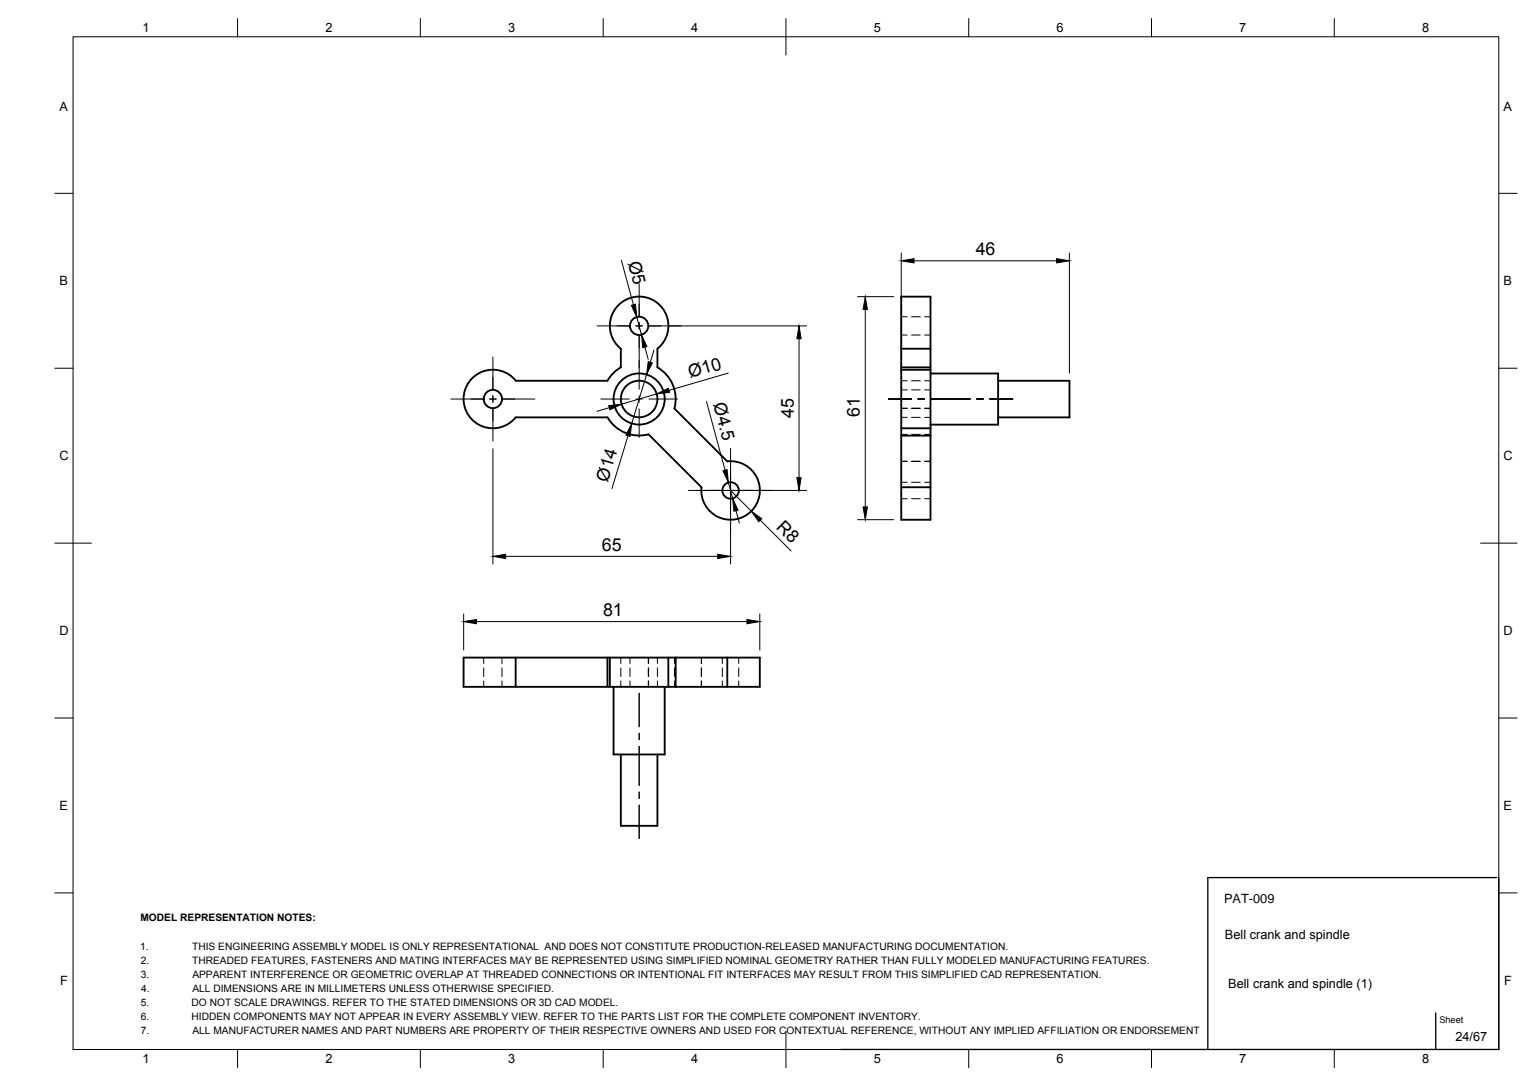
ISO-10303-21;
HEADER;
/* Generated by software containing ST-Developer
 * from STEP Tools, Inc. (www.steptools.com) 
 */

FILE_DESCRIPTION(
/* description */ ('Bell-crank linkage with push rods'),
/* implementation_level */ '2;1');

FILE_NAME(
/* name */ 'Bell crank and spindle (1).step',
/* time_stamp */ '2026-10-28T03:25:15-07:00',
/* author */ (''),
/* organization */ (''),
/* preprocessor_version */ 'ST-DEVELOPER v20.2',
/* originating_system */ 'Autodesk Translation Framework v15.17.0.0',
/* authorisation */ '');

FILE_SCHEMA (('AUTOMOTIVE_DESIGN { 1 0 10303 214 3 1 1 }'));
ENDSEC;

DATA;
#10=MECHANICAL_DESIGN_GEOMETRIC_PRESENTATION_REPRESENTATION('',(#629),#16678);
#513=SHAPE_REPRESENTATION_RELATIONSHIP('SRR','None',#16931,#567);
#567=ADVANCED_BREP_SHAPE_REPRESENTATION('',(#690),#16636);
#629=STYLED_ITEM('',(#17284),#690);
#690=MANIFOLD_SOLID_BREP('Body1',#8820);
#823=FACE_BOUND('',#2103,.T.);
#824=FACE_BOUND('',#2104,.T.);
#825=FACE_BOUND('',#2105,.T.);
#826=FACE_BOUND('',#2112,.T.);
#827=FACE_BOUND('',#2113,.T.);
#828=FACE_BOUND('',#2114,.T.);
#829=FACE_BOUND('',#2115,.T.);
#830=FACE_BOUND('',#2122,.T.);
#1082=PLANE('',#9961);
#1083=PLANE('',#9962);
#1084=PLANE('',#9968);
#1085=PLANE('',#9975);
#1086=PLANE('',#9976);
#1087=PLANE('',#9980);
#1088=PLANE('',#9982);
#1089=PLANE('',#9983);
#1090=PLANE('',#9985);
#1091=PLANE('',#9991);
#1477=FACE_OUTER_BOUND('',#2097,.T.);
#1478=FACE_OUTER_BOUND('',#2098,.T.);
#1479=FACE_OUTER_BOUND('',#2099,.T.);
#1480=FACE_OUTER_BOUND('',#2100,.T.);
#1481=FACE_OUTER_BOUND('',#2101,.T.);
#1482=FACE_OUTER_BOUND('',#2102,.T.);
#1483=FACE_OUTER_BOUND('',#2106,.T.);
#1484=FACE_OUTER_BOUND('',#2107,.T.);
#1485=FACE_OUTER_BOUND('',#2108,.T.);
#1486=FACE_OUTER_BOUND('',#2109,.T.);
#1487=FACE_OUTER_BOUND('',#2110,.T.);
#1488=FACE_OUTER_BOUND('',#2111,.T.);
#1489=FACE_OUTER_BOUND('',#2116,.T.);
#1490=FACE_OUTER_BOUND('',#2117,.T.);
#1491=FACE_OUTER_BOUND('',#2118,.T.);
#1492=FACE_OUTER_BOUND('',#2119,.T.);
#1493=FACE_OUTER_BOUND('',#2120,.T.);
#1494=FACE_OUTER_BOUND('',#2121,.T.);
#1495=FACE_OUTER_BOUND('',#2123,.T.);
#1496=FACE_OUTER_BOUND('',#2124,.T.);
#1497=FACE_OUTER_BOUND('',#2125,.T.);
#2097=EDGE_LOOP('',(#6947,#6948,#6949,#6950));
#2098=EDGE_LOOP('',(#6951,#6952,#6953,#6954));
#2099=EDGE_LOOP('',(#6955,#6956,#6957,#6958));
#2100=EDGE_LOOP('',(#6959,#6960,#6961,#6962));
#2101=EDGE_LOOP('',(#6963,#6964,#6965,#6966));
#2102=EDGE_LOOP('',(#6967,#6968,#6969,#6970,#6971,#6972,#6973,#6974,#6975,
#6976,#6977,#6978));
#2103=EDGE_LOOP('',(#6979));
#2104=EDGE_LOOP('',(#6980));
#2105=EDGE_LOOP('',(#6981));
#2106=EDGE_LOOP('',(#6982,#6983,#6984,#6985));
#2107=EDGE_LOOP('',(#6986,#6987,#6988,#6989));
#2108=EDGE_LOOP('',(#6990,#6991,#6992,#6993));
#2109=EDGE_LOOP('',(#6994,#6995,#6996,#6997));
#2110=EDGE_LOOP('',(#6998,#6999,#7000,#7001));
#2111=EDGE_LOOP('',(#7002,#7003,#7004,#7005,#7006,#7007,#7008,#7009,#7010,
#7011,#7012,#7013));
#2112=EDGE_LOOP('',(#7014));
#2113=EDGE_LOOP('',(#7015));
#2114=EDGE_LOOP('',(#7016));
#2115=EDGE_LOOP('',(#7017));
#2116=EDGE_LOOP('',(#7018,#7019,#7020,#7021));
#2117=EDGE_LOOP('',(#7022,#7023,#7024,#7025));
#2118=EDGE_LOOP('',(#7026,#7027,#7028,#7029));
#2119=EDGE_LOOP('',(#7030,#7031,#7032,#7033));
#2120=EDGE_LOOP('',(#7034,#7035,#7036,#7037));
#2121=EDGE_LOOP('',(#7038));
#2122=EDGE_LOOP('',(#7039));
#2123=EDGE_LOOP('',(#7040,#7041,#7042,#7043));
#2124=EDGE_LOOP('',(#7044,#7045,#7046,#7047));
#2125=EDGE_LOOP('',(#7048));
#2778=LINE('',#15134,#3327);
#2779=LINE('',#15140,#3328);
#2780=LINE('',#15146,#3329);
#2781=LINE('',#15151,#3330);
#2782=LINE('',#15155,#3331);
#2783=LINE('',#15159,#3332);
#2784=LINE('',#15161,#3333);
#2785=LINE('',#15162,#3334);
#2786=LINE('',#15165,#3335);
#2787=LINE('',#15169,#3336);
#2788=LINE('',#15173,#3337);
#2789=LINE('',#15177,#3338);
#2790=LINE('',#15181,#3339);
#2791=LINE('',#15185,#3340);
#2792=LINE('',#15186,#3341);
#2793=LINE('',#15189,#3342);
#2794=LINE('',#15194,#3343);
#2795=LINE('',#15197,#3344);
#2796=LINE('',#15199,#3345);
#2797=LINE('',#15203,#3346);
#2798=LINE('',#15204,#3347);
#2799=LINE('',#15207,#3348);
#2800=LINE('',#15211,#3349);
#2801=LINE('',#15213,#3350);
#2802=LINE('',#15218,#3351);
#2803=LINE('',#15219,#3352);
#2804=LINE('',#15221,#3353);
#2805=LINE('',#15230,#3354);
#2806=LINE('',#15233,#3355);
#3327=VECTOR('',#11870,0.25);
#3328=VECTOR('',#11877,0.25);
#3329=VECTOR('',#11884,0.225);
#3330=VECTOR('',#11889,1.);
#3331=VECTOR('',#11892,1.);
#3332=VECTOR('',#11897,1.);
#3333=VECTOR('',#11898,1.);
#3334=VECTOR('',#11899,1.);
#3335=VECTOR('',#11902,1.);
#3336=VECTOR('',#11905,1.);
#3337=VECTOR('',#11908,1.);
#3338=VECTOR('',#11911,1.);
#3339=VECTOR('',#11914,1.);
#3340=VECTOR('',#11919,1.);
#3341=VECTOR('',#11920,1.);
#3342=VECTOR('',#11923,1.);
#3343=VECTOR('',#11930,1.);
#3344=VECTOR('',#11933,1.);
#3345=VECTOR('',#11934,1.);
#3346=VECTOR('',#11939,1.);
#3347=VECTOR('',#11940,1.);
#3348=VECTOR('',#11943,1.);
#3349=VECTOR('',#11946,1.);
#3350=VECTOR('',#11949,1.);
#3351=VECTOR('',#11956,1.);
#3352=VECTOR('',#11957,1.);
#3353=VECTOR('',#11960,1.);
#3354=VECTOR('',#11973,0.7);
#3355=VECTOR('',#11976,0.5);
#3868=CIRCLE('',#9950,0.25);
#3869=CIRCLE('',#9951,0.25);
#3870=CIRCLE('',#9953,0.25);
#3871=CIRCLE('',#9954,0.25);
#3872=CIRCLE('',#9956,0.225);
#3873=CIRCLE('',#9957,0.225);
#3874=CIRCLE('',#9959,0.8);
#3875=CIRCLE('',#9960,0.8);
#3876=CIRCLE('',#9963,1.);
#3877=CIRCLE('',#9964,0.8);
#3878=CIRCLE('',#9965,1.);
#3879=CIRCLE('',#9966,0.8);
#3880=CIRCLE('',#9967,1.);
#3881=CIRCLE('',#9970,1.);
#3882=CIRCLE('',#9972,1.);
#3883=CIRCLE('',#9974,0.8);
#3884=CIRCLE('',#9977,0.8);
#3885=CIRCLE('',#9978,1.);
#3886=CIRCLE('',#9979,0.7);
#3887=CIRCLE('',#9986,0.7);
#3888=CIRCLE('',#9987,0.5);
#3889=CIRCLE('',#9990,0.5);
#4462=VERTEX_POINT('',#15131);
#4463=VERTEX_POINT('',#15133);
#4464=VERTEX_POINT('',#15137);
#4465=VERTEX_POINT('',#15139);
#4466=VERTEX_POINT('',#15143);
#4467=VERTEX_POINT('',#15145);
#4468=VERTEX_POINT('',#15149);
#4469=VERTEX_POINT('',#15150);
#4470=VERTEX_POINT('',#15152);
#4471=VERTEX_POINT('',#15154);
#4472=VERTEX_POINT('',#15158);
#4473=VERTEX_POINT('',#15160);
#4474=VERTEX_POINT('',#15164);
#4475=VERTEX_POINT('',#15166);
#4476=VERTEX_POINT('',#15168);
#4477=VERTEX_POINT('',#15170);
#4478=VERTEX_POINT('',#15172);
#4479=VERTEX_POINT('',#15174);
#4480=VERTEX_POINT('',#15176);
#4481=VERTEX_POINT('',#15178);
#4482=VERTEX_POINT('',#15180);
#4483=VERTEX_POINT('',#15184);
#4484=VERTEX_POINT('',#15188);
#4485=VERTEX_POINT('',#15192);
#4486=VERTEX_POINT('',#15196);
#4487=VERTEX_POINT('',#15198);
#4488=VERTEX_POINT('',#15202);
#4489=VERTEX_POINT('',#15206);
#4490=VERTEX_POINT('',#15208);
#4491=VERTEX_POINT('',#15210);
#4492=VERTEX_POINT('',#15214);
#4493=VERTEX_POINT('',#15225);
#4494=VERTEX_POINT('',#15227);
#4495=VERTEX_POINT('',#15232);
#5351=EDGE_CURVE('',#4462,#4462,#3868,.T.);
#5352=EDGE_CURVE('',#4462,#4463,#2778,.T.);
#5353=EDGE_CURVE('',#4463,#4463,#3869,.T.);
#5354=EDGE_CURVE('',#4464,#4464,#3870,.T.);
#5355=EDGE_CURVE('',#4464,#4465,#2779,.T.);
#5356=EDGE_CURVE('',#4465,#4465,#3871,.T.);
#5357=EDGE_CURVE('',#4466,#4466,#3872,.T.);
#5358=EDGE_CURVE('',#4466,#4467,#2780,.T.);
#5359=EDGE_CURVE('',#4467,#4467,#3873,.T.);
#5360=EDGE_CURVE('',#4468,#4469,#2781,.T.);
#5361=EDGE_CURVE('',#4468,#4470,#3874,.T.);
#5362=EDGE_CURVE('',#4471,#4470,#2782,.T.);
#5363=EDGE_CURVE('',#4469,#4471,#3875,.T.);
#5364=EDGE_CURVE('',#4472,#4469,#2783,.T.);
#5365=EDGE_CURVE('',#4473,#4472,#2784,.T.);
#5366=EDGE_CURVE('',#4468,#4473,#2785,.T.);
#5367=EDGE_CURVE('',#4471,#4474,#2786,.T.);
#5368=EDGE_CURVE('',#4474,#4475,#3876,.T.);
#5369=EDGE_CURVE('',#4475,#4476,#2787,.T.);
#5370=EDGE_CURVE('',#4476,#4477,#3877,.T.);
#5371=EDGE_CURVE('',#4477,#4478,#2788,.T.);
#5372=EDGE_CURVE('',#4478,#4479,#3878,.T.);
#5373=EDGE_CURVE('',#4479,#4480,#2789,.T.);
#5374=EDGE_CURVE('',#4480,#4481,#3879,.T.);
#5375=EDGE_CURVE('',#4481,#4482,#2790,.T.);
#5376=EDGE_CURVE('',#4482,#4472,#3880,.T.);
#5377=EDGE_CURVE('',#4483,#4470,#2791,.T.);
#5378=EDGE_CURVE('',#4474,#4483,#2792,.T.);
#5379=EDGE_CURVE('',#4482,#4484,#2793,.T.);
#5380=EDGE_CURVE('',#4484,#4473,#3881,.T.);
#5381=EDGE_CURVE('',#4483,#4485,#3882,.T.);
#5382=EDGE_CURVE('',#4485,#4475,#2794,.T.);
#5383=EDGE_CURVE('',#4477,#4486,#2795,.T.);
#5384=EDGE_CURVE('',#4487,#4476,#2796,.T.);
#5385=EDGE_CURVE('',#4487,#4486,#3883,.T.);
#5386=EDGE_CURVE('',#4488,#4486,#2797,.T.);
#5387=EDGE_CURVE('',#4478,#4488,#2798,.T.);
#5388=EDGE_CURVE('',#4484,#4489,#2799,.T.);
#5389=EDGE_CURVE('',#4490,#4489,#3884,.T.);
#5390=EDGE_CURVE('',#4490,#4491,#2800,.T.);
#5391=EDGE_CURVE('',#4488,#4491,#3885,.T.);
#5392=EDGE_CURVE('',#4487,#4485,#2801,.T.);
#5393=EDGE_CURVE('',#4492,#4492,#3886,.T.);
#5394=EDGE_CURVE('',#4490,#4480,#2802,.T.);
#5395=EDGE_CURVE('',#4481,#4489,#2803,.T.);
#5396=EDGE_CURVE('',#4491,#4479,#2804,.T.);
#5397=EDGE_CURVE('',#4493,#4493,#3887,.T.);
#5398=EDGE_CURVE('',#4494,#4494,#3888,.T.);
#5399=EDGE_CURVE('',#4492,#4493,#2805,.T.);
#5400=EDGE_CURVE('',#4494,#4495,#2806,.T.);
#5401=EDGE_CURVE('',#4495,#4495,#3889,.T.);
#6947=ORIENTED_EDGE('',*,*,#5351,.F.);
#6948=ORIENTED_EDGE('',*,*,#5352,.T.);
#6949=ORIENTED_EDGE('',*,*,#5353,.F.);
#6950=ORIENTED_EDGE('',*,*,#5352,.F.);
#6951=ORIENTED_EDGE('',*,*,#5354,.F.);
#6952=ORIENTED_EDGE('',*,*,#5355,.T.);
#6953=ORIENTED_EDGE('',*,*,#5356,.F.);
#6954=ORIENTED_EDGE('',*,*,#5355,.F.);
#6955=ORIENTED_EDGE('',*,*,#5357,.F.);
#6956=ORIENTED_EDGE('',*,*,#5358,.T.);
#6957=ORIENTED_EDGE('',*,*,#5359,.F.);
#6958=ORIENTED_EDGE('',*,*,#5358,.F.);
#6959=ORIENTED_EDGE('',*,*,#5360,.F.);
#6960=ORIENTED_EDGE('',*,*,#5361,.T.);
#6961=ORIENTED_EDGE('',*,*,#5362,.F.);
#6962=ORIENTED_EDGE('',*,*,#5363,.F.);
#6963=ORIENTED_EDGE('',*,*,#5360,.T.);
#6964=ORIENTED_EDGE('',*,*,#5364,.F.);
#6965=ORIENTED_EDGE('',*,*,#5365,.F.);
#6966=ORIENTED_EDGE('',*,*,#5366,.F.);
#6967=ORIENTED_EDGE('',*,*,#5363,.T.);
#6968=ORIENTED_EDGE('',*,*,#5367,.T.);
#6969=ORIENTED_EDGE('',*,*,#5368,.T.);
#6970=ORIENTED_EDGE('',*,*,#5369,.T.);
#6971=ORIENTED_EDGE('',*,*,#5370,.T.);
#6972=ORIENTED_EDGE('',*,*,#5371,.T.);
#6973=ORIENTED_EDGE('',*,*,#5372,.T.);
#6974=ORIENTED_EDGE('',*,*,#5373,.T.);
#6975=ORIENTED_EDGE('',*,*,#5374,.T.);
#6976=ORIENTED_EDGE('',*,*,#5375,.T.);
#6977=ORIENTED_EDGE('',*,*,#5376,.T.);
#6978=ORIENTED_EDGE('',*,*,#5364,.T.);
#6979=ORIENTED_EDGE('',*,*,#5353,.T.);
#6980=ORIENTED_EDGE('',*,*,#5356,.T.);
#6981=ORIENTED_EDGE('',*,*,#5359,.T.);
#6982=ORIENTED_EDGE('',*,*,#5362,.T.);
#6983=ORIENTED_EDGE('',*,*,#5377,.F.);
#6984=ORIENTED_EDGE('',*,*,#5378,.F.);
#6985=ORIENTED_EDGE('',*,*,#5367,.F.);
#6986=ORIENTED_EDGE('',*,*,#5365,.T.);
#6987=ORIENTED_EDGE('',*,*,#5376,.F.);
#6988=ORIENTED_EDGE('',*,*,#5379,.T.);
#6989=ORIENTED_EDGE('',*,*,#5380,.T.);
#6990=ORIENTED_EDGE('',*,*,#5378,.T.);
#6991=ORIENTED_EDGE('',*,*,#5381,.T.);
#6992=ORIENTED_EDGE('',*,*,#5382,.T.);
#6993=ORIENTED_EDGE('',*,*,#5368,.F.);
#6994=ORIENTED_EDGE('',*,*,#5383,.F.);
#6995=ORIENTED_EDGE('',*,*,#5370,.F.);
#6996=ORIENTED_EDGE('',*,*,#5384,.F.);
#6997=ORIENTED_EDGE('',*,*,#5385,.T.);
#6998=ORIENTED_EDGE('',*,*,#5383,.T.);
#6999=ORIENTED_EDGE('',*,*,#5386,.F.);
#7000=ORIENTED_EDGE('',*,*,#5387,.F.);
#7001=ORIENTED_EDGE('',*,*,#5371,.F.);
#7002=ORIENTED_EDGE('',*,*,#5366,.T.);
#7003=ORIENTED_EDGE('',*,*,#5380,.F.);
#7004=ORIENTED_EDGE('',*,*,#5388,.T.);
#7005=ORIENTED_EDGE('',*,*,#5389,.F.);
#7006=ORIENTED_EDGE('',*,*,#5390,.T.);
#7007=ORIENTED_EDGE('',*,*,#5391,.F.);
#7008=ORIENTED_EDGE('',*,*,#5386,.T.);
#7009=ORIENTED_EDGE('',*,*,#5385,.F.);
#7010=ORIENTED_EDGE('',*,*,#5392,.T.);
#7011=ORIENTED_EDGE('',*,*,#5381,.F.);
#7012=ORIENTED_EDGE('',*,*,#5377,.T.);
#7013=ORIENTED_EDGE('',*,*,#5361,.F.);
#7014=ORIENTED_EDGE('',*,*,#5351,.T.);
#7015=ORIENTED_EDGE('',*,*,#5354,.T.);
#7016=ORIENTED_EDGE('',*,*,#5357,.T.);
#7017=ORIENTED_EDGE('',*,*,#5393,.T.);
#7018=ORIENTED_EDGE('',*,*,#5384,.T.);
#7019=ORIENTED_EDGE('',*,*,#5369,.F.);
#7020=ORIENTED_EDGE('',*,*,#5382,.F.);
#7021=ORIENTED_EDGE('',*,*,#5392,.F.);
#7022=ORIENTED_EDGE('',*,*,#5394,.F.);
#7023=ORIENTED_EDGE('',*,*,#5389,.T.);
#7024=ORIENTED_EDGE('',*,*,#5395,.F.);
#7025=ORIENTED_EDGE('',*,*,#5374,.F.);
#7026=ORIENTED_EDGE('',*,*,#5394,.T.);
#7027=ORIENTED_EDGE('',*,*,#5373,.F.);
#7028=ORIENTED_EDGE('',*,*,#5396,.F.);
#7029=ORIENTED_EDGE('',*,*,#5390,.F.);
#7030=ORIENTED_EDGE('',*,*,#5395,.T.);
#7031=ORIENTED_EDGE('',*,*,#5388,.F.);
#7032=ORIENTED_EDGE('',*,*,#5379,.F.);
#7033=ORIENTED_EDGE('',*,*,#5375,.F.);
#7034=ORIENTED_EDGE('',*,*,#5387,.T.);
#7035=ORIENTED_EDGE('',*,*,#5391,.T.);
#7036=ORIENTED_EDGE('',*,*,#5396,.T.);
#7037=ORIENTED_EDGE('',*,*,#5372,.F.);
#7038=ORIENTED_EDGE('',*,*,#5397,.F.);
#7039=ORIENTED_EDGE('',*,*,#5398,.F.);
#7040=ORIENTED_EDGE('',*,*,#5393,.F.);
#7041=ORIENTED_EDGE('',*,*,#5399,.T.);
#7042=ORIENTED_EDGE('',*,*,#5397,.T.);
#7043=ORIENTED_EDGE('',*,*,#5399,.F.);
#7044=ORIENTED_EDGE('',*,*,#5398,.T.);
#7045=ORIENTED_EDGE('',*,*,#5400,.T.);
#7046=ORIENTED_EDGE('',*,*,#5401,.T.);
#7047=ORIENTED_EDGE('',*,*,#5400,.F.);
#7048=ORIENTED_EDGE('',*,*,#5401,.F.);
#8153=CYLINDRICAL_SURFACE('',#9949,0.25);
#8154=CYLINDRICAL_SURFACE('',#9952,0.25);
#8155=CYLINDRICAL_SURFACE('',#9955,0.225);
#8156=CYLINDRICAL_SURFACE('',#9958,0.8);
#8157=CYLINDRICAL_SURFACE('',#9969,1.);
#8158=CYLINDRICAL_SURFACE('',#9971,1.);
#8159=CYLINDRICAL_SURFACE('',#9973,0.8);
#8160=CYLINDRICAL_SURFACE('',#9981,0.8);
#8161=CYLINDRICAL_SURFACE('',#9984,1.);
#8162=CYLINDRICAL_SURFACE('',#9988,0.7);
#8163=CYLINDRICAL_SURFACE('',#9989,0.5);
#8502=ADVANCED_FACE('',(#1477),#8153,.F.);
#8503=ADVANCED_FACE('',(#1478),#8154,.F.);
#8504=ADVANCED_FACE('',(#1479),#8155,.F.);
#8505=ADVANCED_FACE('',(#1480),#8156,.T.);
#8506=ADVANCED_FACE('',(#1481),#1082,.T.);
#8507=ADVANCED_FACE('',(#1482,#823,#824,#825),#1083,.T.);
#8508=ADVANCED_FACE('',(#1483),#1084,.T.);
#8509=ADVANCED_FACE('',(#1484),#8157,.T.);
#8510=ADVANCED_FACE('',(#1485),#8158,.T.);
#8511=ADVANCED_FACE('',(#1486),#8159,.T.);
#8512=ADVANCED_FACE('',(#1487),#1085,.T.);
#8513=ADVANCED_FACE('',(#1488,#826,#827,#828,#829),#1086,.F.);
#8514=ADVANCED_FACE('',(#1489),#1087,.T.);
#8515=ADVANCED_FACE('',(#1490),#8160,.T.);
#8516=ADVANCED_FACE('',(#1491),#1088,.T.);
#8517=ADVANCED_FACE('',(#1492),#1089,.T.);
#8518=ADVANCED_FACE('',(#1493),#8161,.T.);
#8519=ADVANCED_FACE('',(#1494,#830),#1090,.F.);
#8520=ADVANCED_FACE('',(#1495),#8162,.T.);
#8521=ADVANCED_FACE('',(#1496),#8163,.T.);
#8522=ADVANCED_FACE('',(#1497),#1091,.F.);
#8820=CLOSED_SHELL('',(#8502,#8503,#8504,#8505,#8506,#8507,#8508,#8509,
#8510,#8511,#8512,#8513,#8514,#8515,#8516,#8517,#8518,#8519,#8520,#8521,
#8522));
#9948=AXIS2_PLACEMENT_3D('',#15129,#11864,#11865);
#9949=AXIS2_PLACEMENT_3D('',#15130,#11866,#11867);
#9950=AXIS2_PLACEMENT_3D('',#15132,#11868,#11869);
#9951=AXIS2_PLACEMENT_3D('',#15135,#11871,#11872);
#9952=AXIS2_PLACEMENT_3D('',#15136,#11873,#11874);
#9953=AXIS2_PLACEMENT_3D('',#15138,#11875,#11876);
#9954=AXIS2_PLACEMENT_3D('',#15141,#11878,#11879);
#9955=AXIS2_PLACEMENT_3D('',#15142,#11880,#11881);
#9956=AXIS2_PLACEMENT_3D('',#15144,#11882,#11883);
#9957=AXIS2_PLACEMENT_3D('',#15147,#11885,#11886);
#9958=AXIS2_PLACEMENT_3D('',#15148,#11887,#11888);
#9959=AXIS2_PLACEMENT_3D('',#15153,#11890,#11891);
#9960=AXIS2_PLACEMENT_3D('',#15156,#11893,#11894);
#9961=AXIS2_PLACEMENT_3D('',#15157,#11895,#11896);
#9962=AXIS2_PLACEMENT_3D('',#15163,#11900,#11901);
#9963=AXIS2_PLACEMENT_3D('',#15167,#11903,#11904);
#9964=AXIS2_PLACEMENT_3D('',#15171,#11906,#11907);
#9965=AXIS2_PLACEMENT_3D('',#15175,#11909,#11910);
#9966=AXIS2_PLACEMENT_3D('',#15179,#11912,#11913);
#9967=AXIS2_PLACEMENT_3D('',#15182,#11915,#11916);
#9968=AXIS2_PLACEMENT_3D('',#15183,#11917,#11918);
#9969=AXIS2_PLACEMENT_3D('',#15187,#11921,#11922);
#9970=AXIS2_PLACEMENT_3D('',#15190,#11924,#11925);
#9971=AXIS2_PLACEMENT_3D('',#15191,#11926,#11927);
#9972=AXIS2_PLACEMENT_3D('',#15193,#11928,#11929);
#9973=AXIS2_PLACEMENT_3D('',#15195,#11931,#11932);
#9974=AXIS2_PLACEMENT_3D('',#15200,#11935,#11936);
#9975=AXIS2_PLACEMENT_3D('',#15201,#11937,#11938);
#9976=AXIS2_PLACEMENT_3D('',#15205,#11941,#11942);
#9977=AXIS2_PLACEMENT_3D('',#15209,#11944,#11945);
#9978=AXIS2_PLACEMENT_3D('',#15212,#11947,#11948);
#9979=AXIS2_PLACEMENT_3D('',#15215,#11950,#11951);
#9980=AXIS2_PLACEMENT_3D('',#15216,#11952,#11953);
#9981=AXIS2_PLACEMENT_3D('',#15217,#11954,#11955);
#9982=AXIS2_PLACEMENT_3D('',#15220,#11958,#11959);
#9983=AXIS2_PLACEMENT_3D('',#15222,#11961,#11962);
#9984=AXIS2_PLACEMENT_3D('',#15223,#11963,#11964);
#9985=AXIS2_PLACEMENT_3D('',#15224,#11965,#11966);
#9986=AXIS2_PLACEMENT_3D('',#15226,#11967,#11968);
#9987=AXIS2_PLACEMENT_3D('',#15228,#11969,#11970);
#9988=AXIS2_PLACEMENT_3D('',#15229,#11971,#11972);
#9989=AXIS2_PLACEMENT_3D('',#15231,#11974,#11975);
#9990=AXIS2_PLACEMENT_3D('',#15234,#11977,#11978);
#9991=AXIS2_PLACEMENT_3D('',#15235,#11979,#11980);
#11864=DIRECTION('axis',(0.,0.,1.));
#11865=DIRECTION('refdir',(1.,0.,0.));
#11866=DIRECTION('center_axis',(0.,0.,1.));
#11867=DIRECTION('ref_axis',(1.,0.,0.));
#11868=DIRECTION('center_axis',(0.,0.,1.));
#11869=DIRECTION('ref_axis',(1.,0.,0.));
#11870=DIRECTION('',(0.,0.,1.));
#11871=DIRECTION('center_axis',(0.,0.,-1.));
#11872=DIRECTION('ref_axis',(1.,0.,0.));
#11873=DIRECTION('center_axis',(0.,0.,1.));
#11874=DIRECTION('ref_axis',(1.,0.,0.));
#11875=DIRECTION('center_axis',(0.,0.,1.));
#11876=DIRECTION('ref_axis',(1.,0.,0.));
#11877=DIRECTION('',(0.,0.,1.));
#11878=DIRECTION('center_axis',(0.,0.,-1.));
#11879=DIRECTION('ref_axis',(1.,0.,0.));
#11880=DIRECTION('center_axis',(0.,0.,1.));
#11881=DIRECTION('ref_axis',(1.,0.,0.));
#11882=DIRECTION('center_axis',(0.,0.,1.));
#11883=DIRECTION('ref_axis',(1.,0.,0.));
#11884=DIRECTION('',(0.,0.,1.));
#11885=DIRECTION('center_axis',(0.,0.,-1.));
#11886=DIRECTION('ref_axis',(1.,0.,0.));
#11887=DIRECTION('center_axis',(0.,0.,1.));
#11888=DIRECTION('ref_axis',(-0.707106781186548,-0.707106781186547,0.));
#11889=DIRECTION('',(0.,0.,1.));
#11890=DIRECTION('center_axis',(0.,0.,1.));
#11891=DIRECTION('ref_axis',(1.,0.,0.));
#11892=DIRECTION('',(0.,0.,-1.));
#11893=DIRECTION('center_axis',(0.,0.,1.));
#11894=DIRECTION('ref_axis',(1.,0.,0.));
#11895=DIRECTION('center_axis',(-0.707106781186548,0.707106781186548,0.));
#11896=DIRECTION('ref_axis',(-0.707106781186548,-0.707106781186548,0.));
#11897=DIRECTION('',(-0.707106781186548,-0.707106781186548,0.));
#11898=DIRECTION('',(0.,0.,1.));
#11899=DIRECTION('',(0.707106781186548,0.707106781186548,0.));
#11900=DIRECTION('center_axis',(0.,0.,1.));
#11901=DIRECTION('ref_axis',(1.,0.,0.));
#11902=DIRECTION('',(0.707106781186548,0.707106781186548,0.));
#11903=DIRECTION('center_axis',(0.,0.,1.));
#11904=DIRECTION('ref_axis',(1.,0.,0.));
#11905=DIRECTION('',(1.,0.,0.));
#11906=DIRECTION('center_axis',(0.,0.,1.));
#11907=DIRECTION('ref_axis',(1.,0.,0.));
#11908=DIRECTION('',(-1.,0.,0.));
#11909=DIRECTION('center_axis',(0.,0.,1.));
#11910=DIRECTION('ref_axis',(1.,0.,0.));
#11911=DIRECTION('',(0.,1.,0.));
#11912=DIRECTION('center_axis',(0.,0.,1.));
#11913=DIRECTION('ref_axis',(1.,0.,0.));
#11914=DIRECTION('',(0.,-1.,0.));
#11915=DIRECTION('center_axis',(0.,0.,1.));
#11916=DIRECTION('ref_axis',(1.,0.,0.));
#11917=DIRECTION('center_axis',(0.707106781186548,-0.707106781186548,0.));
#11918=DIRECTION('ref_axis',(0.707106781186548,0.707106781186548,0.));
#11919=DIRECTION('',(-0.707106781186548,-0.707106781186548,0.));
#11920=DIRECTION('',(0.,0.,-1.));
#11921=DIRECTION('center_axis',(0.,0.,1.));
#11922=DIRECTION('ref_axis',(-0.923879532511287,0.38268343236509,0.));
#11923=DIRECTION('',(0.,0.,-1.));
#11924=DIRECTION('center_axis',(0.,0.,1.));
#11925=DIRECTION('ref_axis',(1.,0.,0.));
#11926=DIRECTION('center_axis',(0.,0.,1.));
#11927=DIRECTION('ref_axis',(1.,0.,0.));
#11928=DIRECTION('center_axis',(0.,0.,1.));
#11929=DIRECTION('ref_axis',(1.,0.,0.));
#11930=DIRECTION('',(0.,0.,1.));
#11931=DIRECTION('center_axis',(0.,0.,1.));
#11932=DIRECTION('ref_axis',(1.,0.,0.));
#11933=DIRECTION('',(0.,0.,-1.));
#11934=DIRECTION('',(0.,0.,1.));
#11935=DIRECTION('center_axis',(0.,0.,1.));
#11936=DIRECTION('ref_axis',(1.,0.,0.));
#11937=DIRECTION('center_axis',(0.,1.,0.));
#11938=DIRECTION('ref_axis',(-1.,0.,0.));
#11939=DIRECTION('',(1.,0.,0.));
#11940=DIRECTION('',(0.,0.,-1.));
#11941=DIRECTION('center_axis',(0.,0.,1.));
#11942=DIRECTION('ref_axis',(1.,0.,0.));
#11943=DIRECTION('',(0.,1.,0.));
#11944=DIRECTION('center_axis',(0.,0.,1.));
#11945=DIRECTION('ref_axis',(1.,0.,0.));
#11946=DIRECTION('',(0.,-1.,0.));
#11947=DIRECTION('center_axis',(0.,0.,1.));
#11948=DIRECTION('ref_axis',(1.,0.,0.));
#11949=DIRECTION('',(-1.,0.,0.));
#11950=DIRECTION('center_axis',(0.,0.,1.));
#11951=DIRECTION('ref_axis',(1.,0.,0.));
#11952=DIRECTION('center_axis',(0.,-1.,0.));
#11953=DIRECTION('ref_axis',(1.,0.,0.));
#11954=DIRECTION('center_axis',(0.,0.,1.));
#11955=DIRECTION('ref_axis',(6.12323399573677E-17,1.,0.));
#11956=DIRECTION('',(0.,0.,1.));
#11957=DIRECTION('',(0.,0.,-1.));
#11958=DIRECTION('center_axis',(1.,0.,0.));
#11959=DIRECTION('ref_axis',(0.,1.,0.));
#11960=DIRECTION('',(0.,0.,1.));
#11961=DIRECTION('center_axis',(-1.,0.,0.));
#11962=DIRECTION('ref_axis',(0.,-1.,0.));
#11963=DIRECTION('center_axis',(0.,0.,1.));
#11964=DIRECTION('ref_axis',(1.,0.,0.));
#11965=DIRECTION('center_axis',(0.,0.,1.));
#11966=DIRECTION('ref_axis',(1.,0.,0.));
#11967=DIRECTION('center_axis',(0.,0.,1.));
#11968=DIRECTION('ref_axis',(1.,0.,0.));
#11969=DIRECTION('center_axis',(0.,0.,-1.));
#11970=DIRECTION('ref_axis',(1.,0.,0.));
#11971=DIRECTION('center_axis',(0.,0.,1.));
#11972=DIRECTION('ref_axis',(1.,0.,0.));
#11973=DIRECTION('',(0.,0.,-1.));
#11974=DIRECTION('center_axis',(0.,0.,1.));
#11975=DIRECTION('ref_axis',(1.,0.,0.));
#11976=DIRECTION('',(0.,0.,-1.));
#11977=DIRECTION('center_axis',(0.,0.,1.));
#11978=DIRECTION('ref_axis',(1.,0.,0.));
#11979=DIRECTION('center_axis',(0.,0.,1.));
#11980=DIRECTION('ref_axis',(1.,0.,0.));
#15129=CARTESIAN_POINT('',(0.,0.,0.));
#15130=CARTESIAN_POINT('Origin',(4.,0.,4.7));
#15131=CARTESIAN_POINT('',(3.75,-3.06161699786838E-17,4.8));
#15132=CARTESIAN_POINT('Origin',(4.,0.,4.8));
#15133=CARTESIAN_POINT('',(3.75,3.06161699786838E-17,5.6));
#15134=CARTESIAN_POINT('',(3.75,-3.06161699786838E-17,4.7));
#15135=CARTESIAN_POINT('Origin',(4.,0.,5.6));
#15136=CARTESIAN_POINT('Origin',(0.,2.,4.7));
#15137=CARTESIAN_POINT('',(-0.25,2.,4.8));
#15138=CARTESIAN_POINT('Origin',(0.,2.,4.8));
#15139=CARTESIAN_POINT('',(-0.25,2.,5.6));
#15140=CARTESIAN_POINT('',(-0.25,2.,4.7));
#15141=CARTESIAN_POINT('Origin',(0.,2.,5.6));
#15142=CARTESIAN_POINT('Origin',(-2.5,-2.5,4.7));
#15143=CARTESIAN_POINT('',(-2.725,-2.5,4.8));
#15144=CARTESIAN_POINT('Origin',(-2.5,-2.5,4.8));
#15145=CARTESIAN_POINT('',(-2.725,-2.5,5.6));
#15146=CARTESIAN_POINT('',(-2.725,-2.5,4.7));
#15147=CARTESIAN_POINT('Origin',(-2.5,-2.5,5.6));
#15148=CARTESIAN_POINT('Origin',(-2.5,-2.5,4.8));
#15149=CARTESIAN_POINT('',(-2.41196534727688,-1.70485856609033,4.8));
#15150=CARTESIAN_POINT('',(-2.41196534727688,-1.70485856609033,5.6));
#15151=CARTESIAN_POINT('',(-2.41196534727688,-1.70485856609033,4.8));
#15152=CARTESIAN_POINT('',(-1.70485856609033,-2.41196534727688,4.8));
#15153=CARTESIAN_POINT('Origin',(-2.5,-2.5,4.8));
#15154=CARTESIAN_POINT('',(-1.70485856609033,-2.41196534727688,5.6));
#15155=CARTESIAN_POINT('',(-1.70485856609033,-2.41196534727688,4.8));
#15156=CARTESIAN_POINT('Origin',(-2.5,-2.5,5.6));
#15157=CARTESIAN_POINT('Origin',(-0.353553390593274,0.353553390593274,4.8));
#15158=CARTESIAN_POINT('',(-0.965925826289068,-0.25881904510252,5.6));
#15159=CARTESIAN_POINT('',(-2.85355339059327,-2.14644660940673,5.6));
#15160=CARTESIAN_POINT('',(-0.965925826289068,-0.258819045102521,4.8));
#15161=CARTESIAN_POINT('',(-0.965925826289068,-0.258819045102521,4.8));
#15162=CARTESIAN_POINT('',(-2.85355339059327,-2.14644660940673,4.8));
#15163=CARTESIAN_POINT('Origin',(0.,0.,5.6));
#15164=CARTESIAN_POINT('',(-0.258819045102521,-0.965925826289068,5.6));
#15165=CARTESIAN_POINT('',(0.353553390593274,-0.353553390593274,5.6));
#15166=CARTESIAN_POINT('',(0.866025403784439,-0.5,5.6));
#15167=CARTESIAN_POINT('Origin',(0.,0.,5.6));
#15168=CARTESIAN_POINT('',(3.37550020016016,-0.5,5.6));
#15169=CARTESIAN_POINT('',(4.,-0.5,5.6));
#15170=CARTESIAN_POINT('',(3.37550020016016,0.5,5.6));
#15171=CARTESIAN_POINT('Origin',(4.,0.,5.6));
#15172=CARTESIAN_POINT('',(0.866025403784439,0.5,5.6));
#15173=CARTESIAN_POINT('',(0.,0.5,5.6));
#15174=CARTESIAN_POINT('',(0.5,0.866025403784439,5.6));
#15175=CARTESIAN_POINT('Origin',(0.,0.,5.6));
#15176=CARTESIAN_POINT('',(0.5,1.37550020016016,5.6));
#15177=CARTESIAN_POINT('',(0.5,2.,5.6));
#15178=CARTESIAN_POINT('',(-0.5,1.37550020016016,5.6));
#15179=CARTESIAN_POINT('Origin',(0.,2.,5.6));
#15180=CARTESIAN_POINT('',(-0.5,0.866025403784439,5.6));
#15181=CARTESIAN_POINT('',(-0.5,0.,5.6));
#15182=CARTESIAN_POINT('Origin',(0.,0.,5.6));
#15183=CARTESIAN_POINT('Origin',(-2.14644660940673,-2.85355339059327,4.8));
#15184=CARTESIAN_POINT('',(-0.25881904510252,-0.965925826289068,4.8));
#15185=CARTESIAN_POINT('',(0.353553390593274,-0.353553390593274,4.8));
#15186=CARTESIAN_POINT('',(-0.25881904510252,-0.965925826289068,4.8));
#15187=CARTESIAN_POINT('Origin',(0.,0.,4.8));
#15188=CARTESIAN_POINT('',(-0.5,0.866025403784439,4.8));
#15189=CARTESIAN_POINT('',(-0.5,0.866025403784439,4.8));
#15190=CARTESIAN_POINT('Origin',(0.,0.,4.8));
#15191=CARTESIAN_POINT('Origin',(0.,0.,4.8));
#15192=CARTESIAN_POINT('',(0.866025403784439,-0.5,4.8));
#15193=CARTESIAN_POINT('Origin',(0.,0.,4.8));
#15194=CARTESIAN_POINT('',(0.866025403784439,-0.5,4.8));
#15195=CARTESIAN_POINT('Origin',(4.,0.,4.8));
#15196=CARTESIAN_POINT('',(3.37550020016016,0.5,4.8));
#15197=CARTESIAN_POINT('',(3.37550020016016,0.5,4.8));
#15198=CARTESIAN_POINT('',(3.37550020016016,-0.5,4.8));
#15199=CARTESIAN_POINT('',(3.37550020016016,-0.5,4.8));
#15200=CARTESIAN_POINT('Origin',(4.,0.,4.8));
#15201=CARTESIAN_POINT('Origin',(4.,0.5,4.8));
#15202=CARTESIAN_POINT('',(0.866025403784439,0.5,4.8));
#15203=CARTESIAN_POINT('',(0.,0.5,4.8));
#15204=CARTESIAN_POINT('',(0.866025403784439,0.5,4.8));
#15205=CARTESIAN_POINT('Origin',(0.,0.,4.8));
#15206=CARTESIAN_POINT('',(-0.5,1.37550020016016,4.8));
#15207=CARTESIAN_POINT('',(-0.5,0.,4.8));
#15208=CARTESIAN_POINT('',(0.5,1.37550020016016,4.8));
#15209=CARTESIAN_POINT('Origin',(0.,2.,4.8));
#15210=CARTESIAN_POINT('',(0.5,0.866025403784439,4.8));
#15211=CARTESIAN_POINT('',(0.5,2.,4.8));
#15212=CARTESIAN_POINT('Origin',(0.,0.,4.8));
#15213=CARTESIAN_POINT('',(4.,-0.5,4.8));
#15214=CARTESIAN_POINT('',(-0.7,-8.57252759403147E-17,4.8));
#15215=CARTESIAN_POINT('Origin',(0.,0.,4.8));
#15216=CARTESIAN_POINT('Origin',(0.,-0.5,4.8));
#15217=CARTESIAN_POINT('Origin',(0.,2.,4.8));
#15218=CARTESIAN_POINT('',(0.5,1.37550020016016,4.8));
#15219=CARTESIAN_POINT('',(-0.5,1.37550020016016,4.8));
#15220=CARTESIAN_POINT('Origin',(0.5,0.,4.8));
#15221=CARTESIAN_POINT('',(0.5,0.866025403784439,4.8));
#15222=CARTESIAN_POINT('Origin',(-0.5,2.,4.8));
#15223=CARTESIAN_POINT('Origin',(0.,0.,4.8));
#15224=CARTESIAN_POINT('Origin',(0.,0.,2.95));
#15225=CARTESIAN_POINT('',(-0.7,-8.57252759403147E-17,2.95));
#15226=CARTESIAN_POINT('Origin',(0.,0.,2.95));
#15227=CARTESIAN_POINT('',(-0.5,6.12323399573677E-17,2.95));
#15228=CARTESIAN_POINT('Origin',(0.,0.,2.95));
#15229=CARTESIAN_POINT('Origin',(0.,0.,2.95));
#15230=CARTESIAN_POINT('',(-0.7,-8.57252759403147E-17,2.95));
#15231=CARTESIAN_POINT('Origin',(0.,0.,1.));
#15232=CARTESIAN_POINT('',(-0.5,-6.12323399573677E-17,1.));
#15233=CARTESIAN_POINT('',(-0.5,-6.12323399573677E-17,1.));
#15234=CARTESIAN_POINT('Origin',(0.,0.,1.));
#15235=CARTESIAN_POINT('Origin',(0.,0.,1.));
#16572=UNCERTAINTY_MEASURE_WITH_UNIT(LENGTH_MEASURE(0.001),#16679,
'DISTANCE_ACCURACY_VALUE',
'Maximum model space distance between geometric entities at asserted c
onnectivities');
#16614=UNCERTAINTY_MEASURE_WITH_UNIT(LENGTH_MEASURE(0.001),#16679,
'DISTANCE_ACCURACY_VALUE',
'Maximum model space distance between geometric entities at asserted c
onnectivities');
#16636=(
GEOMETRIC_REPRESENTATION_CONTEXT(3)
GLOBAL_UNCERTAINTY_ASSIGNED_CONTEXT((#16572))
GLOBAL_UNIT_ASSIGNED_CONTEXT((#16679,#16681,#16682))
REPRESENTATION_CONTEXT('','3D')
);
#16678=(
GEOMETRIC_REPRESENTATION_CONTEXT(3)
GLOBAL_UNCERTAINTY_ASSIGNED_CONTEXT((#16614))
GLOBAL_UNIT_ASSIGNED_CONTEXT((#16679,#16681,#16682))
REPRESENTATION_CONTEXT('','3D')
);
#16679=(
LENGTH_UNIT()
NAMED_UNIT(*)
SI_UNIT(.CENTI.,.METRE.)
);
#16681=(
NAMED_UNIT(*)
PLANE_ANGLE_UNIT()
SI_UNIT($,.RADIAN.)
);
#16682=(
NAMED_UNIT(*)
SI_UNIT($,.STERADIAN.)
SOLID_ANGLE_UNIT()
);
#16704=SHAPE_DEFINITION_REPRESENTATION(#16772,#16931);
#16772=PRODUCT_DEFINITION_SHAPE('',$,#16995);
#16931=SHAPE_REPRESENTATION('',(#9948),#16636);
#16973=PRODUCT_DEFINITION_CONTEXT('part definition',#17164,'design');
#16995=PRODUCT_DEFINITION('Bell crank and spindle (1)',
'Bell crank and spindle (1)',#17058,#16973);
#17058=PRODUCT_DEFINITION_FORMATION('',$,#17187);
#17164=APPLICATION_CONTEXT(
'Core Data for Automotive Mechanical Design Process');
#17165=PRODUCT_CONTEXT('part definition',#17164,'mechanical');
#17187=PRODUCT('Bell crank and spindle (1)','Bell crank and spindle (1)',
'Bell crank and spindle (1)',(#17165));
#17278=COLOUR_RGB('Sky Blue',0.24,0.69,0.87);
#17279=FILL_AREA_STYLE_COLOUR('',#17278);
#17280=FILL_AREA_STYLE('',(#17279));
#17281=SURFACE_STYLE_FILL_AREA(#17280);
#17282=SURFACE_SIDE_STYLE('',(#17281));
#17283=SURFACE_STYLE_USAGE(.BOTH.,#17282);
#17284=PRESENTATION_STYLE_ASSIGNMENT((#17283));
ENDSEC;
END-ISO-10303-21;
